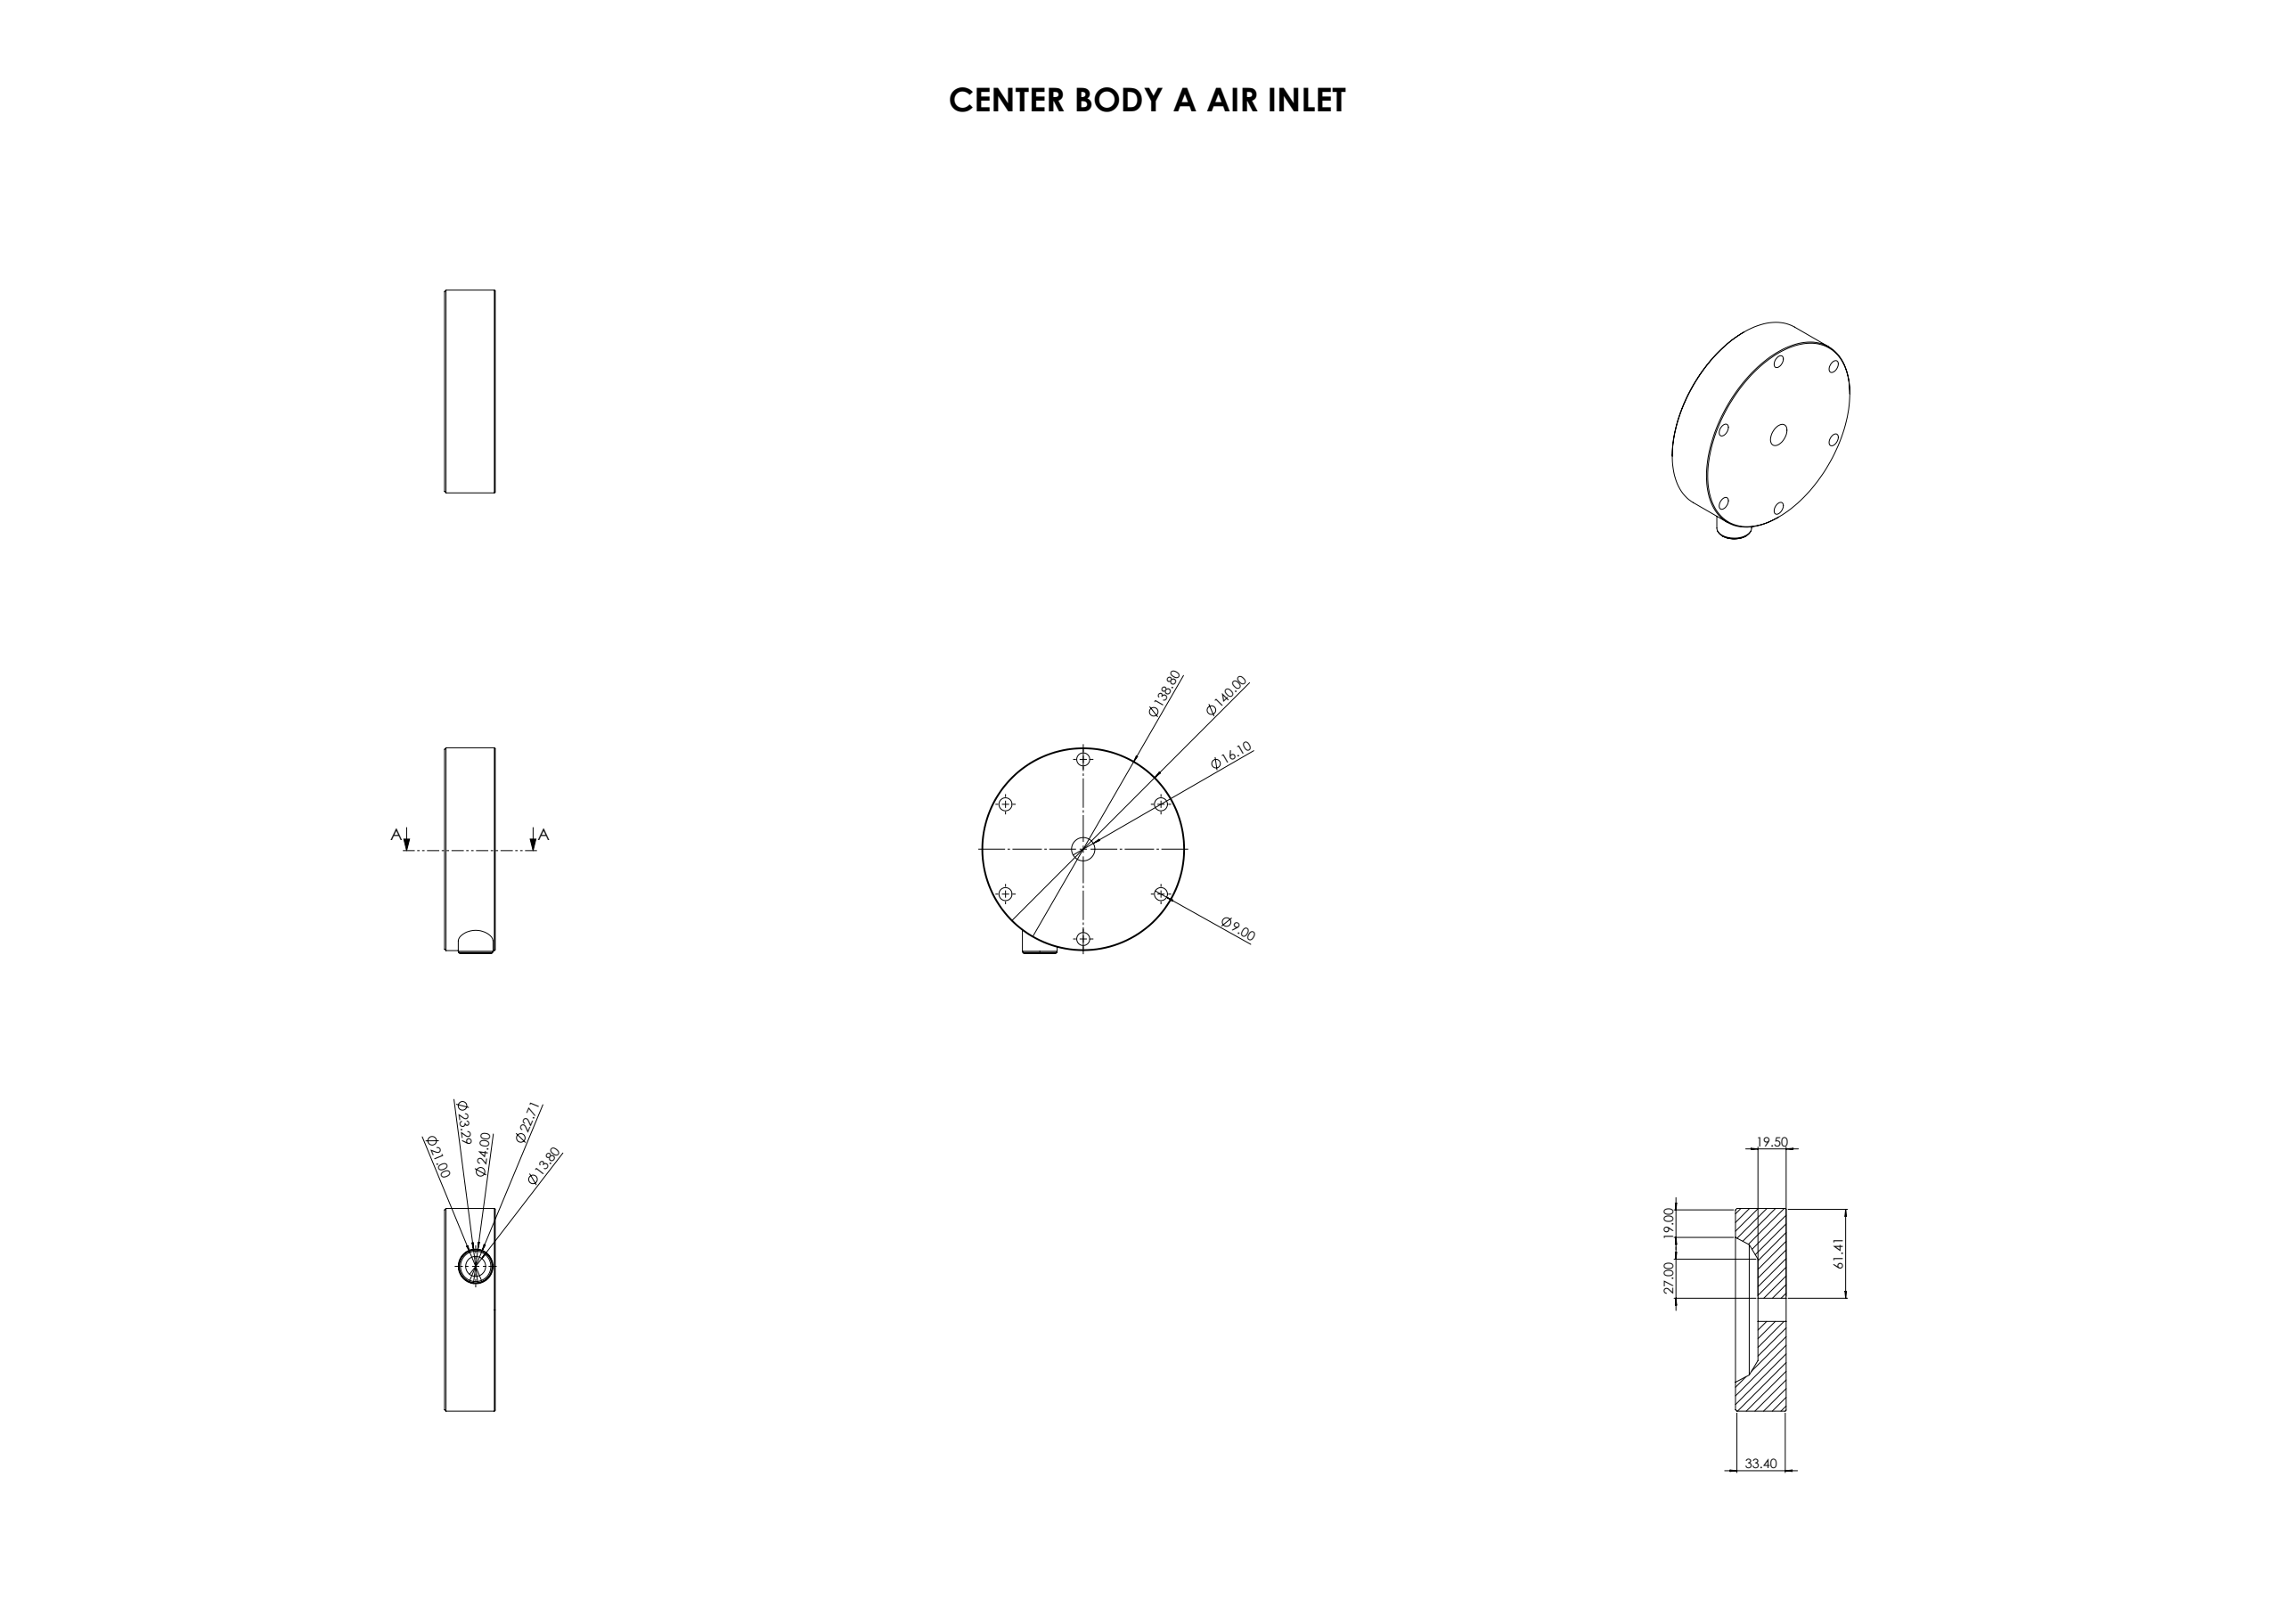
ISO-10303-21;
HEADER;
/* Generated by software containing ST-Developer
 * from STEP Tools, Inc. (www.steptools.com) 
 */

FILE_DESCRIPTION(
/* description */ (''),
/* implementation_level */ '2;1');

FILE_NAME(
/* name */ '02_Center_Body_A_Air_Inlet.step',
/* time_stamp */ '2026-10-26T06:13:19-07:00',
/* author */ (''),
/* organization */ (''),
/* preprocessor_version */ 'ST-DEVELOPER v20.2',
/* originating_system */ 'Autodesk Translation Framework v15.15.0.0',
/* authorisation */ '');

FILE_SCHEMA (('AUTOMOTIVE_DESIGN { 1 0 10303 214 3 1 1 }','TECHNICAL_DATA_PACKAGING'));
ENDSEC;

DATA;
#10=MECHANICAL_DESIGN_GEOMETRIC_PRESENTATION_REPRESENTATION('',(#298),#56639);
#258=SHAPE_REPRESENTATION_RELATIONSHIP('SRR','None',#56746,#278);
#278=ADVANCED_BREP_SHAPE_REPRESENTATION('',(#318),#56620);
#298=STYLED_ITEM('',(#56894),#318);
#318=MANIFOLD_SOLID_BREP('Body1',#16950);
#442=FACE_BOUND('',#2951,.T.);
#443=FACE_BOUND('',#2956,.T.);
#444=FACE_BOUND('',#2958,.T.);
#445=FACE_BOUND('',#2959,.T.);
#446=FACE_BOUND('',#2960,.T.);
#447=FACE_BOUND('',#2961,.T.);
#448=FACE_BOUND('',#2962,.T.);
#449=FACE_BOUND('',#2963,.T.);
#450=FACE_BOUND('',#2964,.T.);
#451=FACE_BOUND('',#2974,.T.);
#452=FACE_BOUND('',#2978,.T.);
#453=FACE_BOUND('',#2979,.T.);
#454=FACE_BOUND('',#2980,.T.);
#455=FACE_BOUND('',#2981,.T.);
#456=FACE_BOUND('',#2982,.T.);
#457=FACE_BOUND('',#2983,.T.);
#458=FACE_BOUND('',#2984,.T.);
#573=CONICAL_SURFACE('',#17486,10.9267766952966,1.17809724509617);
#574=CONICAL_SURFACE('',#17489,11.5,0.785398163397449);
#575=CONICAL_SURFACE('',#17493,11.8232233047034,0.392699081698727);
#576=CONICAL_SURFACE('',#17496,69.7,0.785398163397444);
#577=CONICAL_SURFACE('',#17528,40.,1.03037682652431);
#578=CONICAL_SURFACE('',#17530,47.5,0.484477929037023);
#579=CONICAL_SURFACE('',#17534,69.5,0.785398163397448);
#815=CIRCLE('',#17487,11.3535533905933);
#816=CIRCLE('',#17488,10.5);
#817=CIRCLE('',#17490,11.6464466094067);
#818=CIRCLE('',#17492,6.9);
#819=CIRCLE('',#17494,12.);
#820=CIRCLE('',#17497,69.4);
#821=CIRCLE('',#17498,70.);
#822=CIRCLE('',#17499,70.);
#823=CIRCLE('',#17501,70.);
#824=CIRCLE('',#17503,4.5);
#825=CIRCLE('',#17504,4.5);
#826=CIRCLE('',#17505,4.5);
#827=CIRCLE('',#17506,4.5);
#828=CIRCLE('',#17507,4.5);
#829=CIRCLE('',#17508,4.5);
#830=CIRCLE('',#17509,8.05);
#831=CIRCLE('',#17511,6.9);
#832=CIRCLE('',#17514,4.5);
#833=CIRCLE('',#17516,4.5);
#834=CIRCLE('',#17518,4.5);
#835=CIRCLE('',#17520,4.5);
#836=CIRCLE('',#17522,4.5);
#837=CIRCLE('',#17524,4.5);
#838=CIRCLE('',#17526,35.);
#839=CIRCLE('',#17527,8.05);
#840=CIRCLE('',#17529,45.);
#841=CIRCLE('',#17531,50.);
#842=CIRCLE('',#17533,69.);
#1281=CYLINDRICAL_SURFACE('',#17495,12.);
#1282=CYLINDRICAL_SURFACE('',#17500,70.);
#1283=CYLINDRICAL_SURFACE('',#17510,6.9);
#1284=CYLINDRICAL_SURFACE('',#17513,4.5);
#1285=CYLINDRICAL_SURFACE('',#17515,4.5);
#1286=CYLINDRICAL_SURFACE('',#17517,4.5);
#1287=CYLINDRICAL_SURFACE('',#17519,4.5);
#1288=CYLINDRICAL_SURFACE('',#17521,4.5);
#1289=CYLINDRICAL_SURFACE('',#17523,4.5);
#1290=CYLINDRICAL_SURFACE('',#17535,8.05);
#1947=FACE_OUTER_BOUND('',#2948,.T.);
#1948=FACE_OUTER_BOUND('',#2949,.T.);
#1949=FACE_OUTER_BOUND('',#2950,.T.);
#1950=FACE_OUTER_BOUND('',#2952,.T.);
#1951=FACE_OUTER_BOUND('',#2953,.T.);
#1952=FACE_OUTER_BOUND('',#2954,.T.);
#1953=FACE_OUTER_BOUND('',#2955,.T.);
#1954=FACE_OUTER_BOUND('',#2957,.T.);
#1955=FACE_OUTER_BOUND('',#2965,.T.);
#1956=FACE_OUTER_BOUND('',#2966,.T.);
#1957=FACE_OUTER_BOUND('',#2967,.T.);
#1958=FACE_OUTER_BOUND('',#2968,.T.);
#1959=FACE_OUTER_BOUND('',#2969,.T.);
#1960=FACE_OUTER_BOUND('',#2970,.T.);
#1961=FACE_OUTER_BOUND('',#2971,.T.);
#1962=FACE_OUTER_BOUND('',#2972,.T.);
#1963=FACE_OUTER_BOUND('',#2973,.T.);
#1964=FACE_OUTER_BOUND('',#2975,.T.);
#1965=FACE_OUTER_BOUND('',#2976,.T.);
#1966=FACE_OUTER_BOUND('',#2977,.T.);
#1967=FACE_OUTER_BOUND('',#2985,.T.);
#1968=FACE_OUTER_BOUND('',#2986,.T.);
#2948=EDGE_LOOP('',(#11496,#11497,#11498,#11499));
#2949=EDGE_LOOP('',(#11500,#11501,#11502,#11503));
#2950=EDGE_LOOP('',(#11504));
#2951=EDGE_LOOP('',(#11505));
#2952=EDGE_LOOP('',(#11506,#11507,#11508,#11509));
#2953=EDGE_LOOP('',(#11510,#11511,#11512,#11513,#11514));
#2954=EDGE_LOOP('',(#11515,#11516,#11517,#11518,#11519));
#2955=EDGE_LOOP('',(#11520,#11521,#11522,#11523,#11524));
#2956=EDGE_LOOP('',(#11525,#11526));
#2957=EDGE_LOOP('',(#11527));
#2958=EDGE_LOOP('',(#11528));
#2959=EDGE_LOOP('',(#11529));
#2960=EDGE_LOOP('',(#11530));
#2961=EDGE_LOOP('',(#11531));
#2962=EDGE_LOOP('',(#11532));
#2963=EDGE_LOOP('',(#11533));
#2964=EDGE_LOOP('',(#11534));
#2965=EDGE_LOOP('',(#11535,#11536,#11537,#11538));
#2966=EDGE_LOOP('',(#11539));
#2967=EDGE_LOOP('',(#11540,#11541,#11542,#11543));
#2968=EDGE_LOOP('',(#11544,#11545,#11546,#11547));
#2969=EDGE_LOOP('',(#11548,#11549,#11550,#11551));
#2970=EDGE_LOOP('',(#11552,#11553,#11554,#11555));
#2971=EDGE_LOOP('',(#11556,#11557,#11558,#11559));
#2972=EDGE_LOOP('',(#11560,#11561,#11562,#11563));
#2973=EDGE_LOOP('',(#11564));
#2974=EDGE_LOOP('',(#11565));
#2975=EDGE_LOOP('',(#11566,#11567,#11568,#11569));
#2976=EDGE_LOOP('',(#11570,#11571,#11572,#11573));
#2977=EDGE_LOOP('',(#11574));
#2978=EDGE_LOOP('',(#11575));
#2979=EDGE_LOOP('',(#11576));
#2980=EDGE_LOOP('',(#11577));
#2981=EDGE_LOOP('',(#11578));
#2982=EDGE_LOOP('',(#11579));
#2983=EDGE_LOOP('',(#11580));
#2984=EDGE_LOOP('',(#11581));
#2985=EDGE_LOOP('',(#11582,#11583,#11584,#11585));
#2986=EDGE_LOOP('',(#11586,#11587,#11588,#11589));
#4042=LINE('',#24660,#4996);
#4043=LINE('',#24664,#4997);
#4044=LINE('',#24671,#4998);
#4045=LINE('',#24675,#4999);
#4046=LINE('',#24721,#5000);
#4047=LINE('',#24727,#5001);
#4048=LINE('',#24746,#5002);
#4049=LINE('',#24751,#5003);
#4050=LINE('',#24755,#5004);
#4051=LINE('',#24759,#5005);
#4052=LINE('',#24763,#5006);
#4053=LINE('',#24767,#5007);
#4054=LINE('',#24771,#5008);
#4055=LINE('',#24780,#5009);
#4056=LINE('',#24784,#5010);
#4057=LINE('',#24790,#5011);
#4058=LINE('',#24792,#5012);
#4996=VECTOR('',#19526,10.9267766952966);
#4997=VECTOR('',#19531,11.5);
#4998=VECTOR('',#19540,11.8232233047034);
#4999=VECTOR('',#19545,12.);
#5000=VECTOR('',#19550,69.7);
#5001=VECTOR('',#19557,70.);
#5002=VECTOR('',#19578,6.9);
#5003=VECTOR('',#19585,4.5);
#5004=VECTOR('',#19590,4.5);
#5005=VECTOR('',#19595,4.5);
#5006=VECTOR('',#19600,4.5);
#5007=VECTOR('',#19605,4.5);
#5008=VECTOR('',#19610,4.5);
#5009=VECTOR('',#19621,40.);
#5010=VECTOR('',#19626,47.5);
#5011=VECTOR('',#19635,69.5);
#5012=VECTOR('',#19638,8.05);
#5877=B_SPLINE_CURVE_WITH_KNOTS('',3,(#24677,#24678,#24679,#24680,#24681,
#24682,#24683,#24684,#24685,#24686),.UNSPECIFIED.,.F.,.F.,(4,2,2,2,4),(0.,
0.449224301228608,0.898448602457216,1.38616749821439,1.87388639397155),
 .UNSPECIFIED.);
#5878=B_SPLINE_CURVE_WITH_KNOTS('',3,(#24687,#24688,#24689,#24690,#24691,
#24692,#24693,#24694,#24695,#24696,#24697,#24698,#24699,#24700,#24701,#24702,
#24703,#24704,#24705,#24706,#24707,#24708,#24709,#24710,#24711,#24712,#24713,
#24714,#24715,#24716),.UNSPECIFIED.,.F.,.F.,(4,2,2,2,2,2,2,2,2,2,2,2,2,
2,4),(1.87388639397155,2.39804133800567,2.92219628203978,3.37669912288026,
3.6039505433005,3.83120196372073,4.05845338414097,4.28570480456121,4.74020764540168,
5.2643625894358,5.78851753346991,6.27623642922708,6.76395532498425,7.21317962621286,
7.66240392744147),.UNSPECIFIED.);
#6943=VERTEX_POINT('',#24657);
#6944=VERTEX_POINT('',#24659);
#6945=VERTEX_POINT('',#24663);
#6946=VERTEX_POINT('',#24667);
#6947=VERTEX_POINT('',#24670);
#6948=VERTEX_POINT('',#24674);
#6949=VERTEX_POINT('',#24676);
#6950=VERTEX_POINT('',#24718);
#6951=VERTEX_POINT('',#24720);
#6952=VERTEX_POINT('',#24722);
#6953=VERTEX_POINT('',#24726);
#6954=VERTEX_POINT('',#24730);
#6955=VERTEX_POINT('',#24732);
#6956=VERTEX_POINT('',#24734);
#6957=VERTEX_POINT('',#24736);
#6958=VERTEX_POINT('',#24738);
#6959=VERTEX_POINT('',#24740);
#6960=VERTEX_POINT('',#24742);
#6961=VERTEX_POINT('',#24745);
#6962=VERTEX_POINT('',#24750);
#6963=VERTEX_POINT('',#24754);
#6964=VERTEX_POINT('',#24758);
#6965=VERTEX_POINT('',#24762);
#6966=VERTEX_POINT('',#24766);
#6967=VERTEX_POINT('',#24770);
#6968=VERTEX_POINT('',#24774);
#6969=VERTEX_POINT('',#24776);
#6970=VERTEX_POINT('',#24779);
#6971=VERTEX_POINT('',#24783);
#6972=VERTEX_POINT('',#24787);
#8655=EDGE_CURVE('',#6943,#6943,#815,.T.);
#8656=EDGE_CURVE('',#6943,#6944,#4042,.T.);
#8657=EDGE_CURVE('',#6944,#6944,#816,.T.);
#8658=EDGE_CURVE('',#6943,#6945,#4043,.T.);
#8659=EDGE_CURVE('',#6945,#6945,#817,.T.);
#8660=EDGE_CURVE('',#6946,#6946,#818,.T.);
#8661=EDGE_CURVE('',#6945,#6947,#4044,.T.);
#8662=EDGE_CURVE('',#6947,#6947,#819,.T.);
#8663=EDGE_CURVE('',#6947,#6948,#4045,.T.);
#8664=EDGE_CURVE('',#6949,#6948,#5877,.T.);
#8665=EDGE_CURVE('',#6948,#6949,#5878,.T.);
#8666=EDGE_CURVE('',#6950,#6950,#820,.T.);
#8667=EDGE_CURVE('',#6950,#6951,#4046,.T.);
#8668=EDGE_CURVE('',#6951,#6952,#821,.T.);
#8669=EDGE_CURVE('',#6952,#6951,#822,.T.);
#8670=EDGE_CURVE('',#6952,#6953,#4047,.T.);
#8671=EDGE_CURVE('',#6953,#6953,#823,.T.);
#8672=EDGE_CURVE('',#6954,#6954,#824,.T.);
#8673=EDGE_CURVE('',#6955,#6955,#825,.T.);
#8674=EDGE_CURVE('',#6956,#6956,#826,.T.);
#8675=EDGE_CURVE('',#6957,#6957,#827,.T.);
#8676=EDGE_CURVE('',#6958,#6958,#828,.T.);
#8677=EDGE_CURVE('',#6959,#6959,#829,.T.);
#8678=EDGE_CURVE('',#6960,#6960,#830,.T.);
#8679=EDGE_CURVE('',#6946,#6961,#4048,.T.);
#8680=EDGE_CURVE('',#6961,#6961,#831,.T.);
#8681=EDGE_CURVE('',#6954,#6962,#4049,.T.);
#8682=EDGE_CURVE('',#6962,#6962,#832,.T.);
#8683=EDGE_CURVE('',#6955,#6963,#4050,.T.);
#8684=EDGE_CURVE('',#6963,#6963,#833,.T.);
#8685=EDGE_CURVE('',#6956,#6964,#4051,.T.);
#8686=EDGE_CURVE('',#6964,#6964,#834,.T.);
#8687=EDGE_CURVE('',#6957,#6965,#4052,.T.);
#8688=EDGE_CURVE('',#6965,#6965,#835,.T.);
#8689=EDGE_CURVE('',#6958,#6966,#4053,.T.);
#8690=EDGE_CURVE('',#6966,#6966,#836,.T.);
#8691=EDGE_CURVE('',#6959,#6967,#4054,.T.);
#8692=EDGE_CURVE('',#6967,#6967,#837,.T.);
#8693=EDGE_CURVE('',#6968,#6968,#838,.T.);
#8694=EDGE_CURVE('',#6969,#6969,#839,.T.);
#8695=EDGE_CURVE('',#6968,#6970,#4055,.T.);
#8696=EDGE_CURVE('',#6970,#6970,#840,.T.);
#8697=EDGE_CURVE('',#6970,#6971,#4056,.T.);
#8698=EDGE_CURVE('',#6971,#6971,#841,.T.);
#8699=EDGE_CURVE('',#6972,#6972,#842,.T.);
#8700=EDGE_CURVE('',#6953,#6972,#4057,.T.);
#8701=EDGE_CURVE('',#6960,#6969,#4058,.T.);
#11496=ORIENTED_EDGE('',*,*,#8655,.T.);
#11497=ORIENTED_EDGE('',*,*,#8656,.T.);
#11498=ORIENTED_EDGE('',*,*,#8657,.T.);
#11499=ORIENTED_EDGE('',*,*,#8656,.F.);
#11500=ORIENTED_EDGE('',*,*,#8655,.F.);
#11501=ORIENTED_EDGE('',*,*,#8658,.T.);
#11502=ORIENTED_EDGE('',*,*,#8659,.F.);
#11503=ORIENTED_EDGE('',*,*,#8658,.F.);
#11504=ORIENTED_EDGE('',*,*,#8657,.F.);
#11505=ORIENTED_EDGE('',*,*,#8660,.T.);
#11506=ORIENTED_EDGE('',*,*,#8659,.T.);
#11507=ORIENTED_EDGE('',*,*,#8661,.T.);
#11508=ORIENTED_EDGE('',*,*,#8662,.T.);
#11509=ORIENTED_EDGE('',*,*,#8661,.F.);
#11510=ORIENTED_EDGE('',*,*,#8662,.F.);
#11511=ORIENTED_EDGE('',*,*,#8663,.T.);
#11512=ORIENTED_EDGE('',*,*,#8664,.F.);
#11513=ORIENTED_EDGE('',*,*,#8665,.F.);
#11514=ORIENTED_EDGE('',*,*,#8663,.F.);
#11515=ORIENTED_EDGE('',*,*,#8666,.T.);
#11516=ORIENTED_EDGE('',*,*,#8667,.T.);
#11517=ORIENTED_EDGE('',*,*,#8668,.T.);
#11518=ORIENTED_EDGE('',*,*,#8669,.T.);
#11519=ORIENTED_EDGE('',*,*,#8667,.F.);
#11520=ORIENTED_EDGE('',*,*,#8668,.F.);
#11521=ORIENTED_EDGE('',*,*,#8669,.F.);
#11522=ORIENTED_EDGE('',*,*,#8670,.T.);
#11523=ORIENTED_EDGE('',*,*,#8671,.T.);
#11524=ORIENTED_EDGE('',*,*,#8670,.F.);
#11525=ORIENTED_EDGE('',*,*,#8664,.T.);
#11526=ORIENTED_EDGE('',*,*,#8665,.T.);
#11527=ORIENTED_EDGE('',*,*,#8666,.F.);
#11528=ORIENTED_EDGE('',*,*,#8672,.T.);
#11529=ORIENTED_EDGE('',*,*,#8673,.T.);
#11530=ORIENTED_EDGE('',*,*,#8674,.T.);
#11531=ORIENTED_EDGE('',*,*,#8675,.T.);
#11532=ORIENTED_EDGE('',*,*,#8676,.T.);
#11533=ORIENTED_EDGE('',*,*,#8677,.T.);
#11534=ORIENTED_EDGE('',*,*,#8678,.F.);
#11535=ORIENTED_EDGE('',*,*,#8660,.F.);
#11536=ORIENTED_EDGE('',*,*,#8679,.T.);
#11537=ORIENTED_EDGE('',*,*,#8680,.T.);
#11538=ORIENTED_EDGE('',*,*,#8679,.F.);
#11539=ORIENTED_EDGE('',*,*,#8680,.F.);
#11540=ORIENTED_EDGE('',*,*,#8672,.F.);
#11541=ORIENTED_EDGE('',*,*,#8681,.T.);
#11542=ORIENTED_EDGE('',*,*,#8682,.F.);
#11543=ORIENTED_EDGE('',*,*,#8681,.F.);
#11544=ORIENTED_EDGE('',*,*,#8673,.F.);
#11545=ORIENTED_EDGE('',*,*,#8683,.T.);
#11546=ORIENTED_EDGE('',*,*,#8684,.F.);
#11547=ORIENTED_EDGE('',*,*,#8683,.F.);
#11548=ORIENTED_EDGE('',*,*,#8674,.F.);
#11549=ORIENTED_EDGE('',*,*,#8685,.T.);
#11550=ORIENTED_EDGE('',*,*,#8686,.F.);
#11551=ORIENTED_EDGE('',*,*,#8685,.F.);
#11552=ORIENTED_EDGE('',*,*,#8675,.F.);
#11553=ORIENTED_EDGE('',*,*,#8687,.T.);
#11554=ORIENTED_EDGE('',*,*,#8688,.F.);
#11555=ORIENTED_EDGE('',*,*,#8687,.F.);
#11556=ORIENTED_EDGE('',*,*,#8676,.F.);
#11557=ORIENTED_EDGE('',*,*,#8689,.T.);
#11558=ORIENTED_EDGE('',*,*,#8690,.F.);
#11559=ORIENTED_EDGE('',*,*,#8689,.F.);
#11560=ORIENTED_EDGE('',*,*,#8677,.F.);
#11561=ORIENTED_EDGE('',*,*,#8691,.T.);
#11562=ORIENTED_EDGE('',*,*,#8692,.F.);
#11563=ORIENTED_EDGE('',*,*,#8691,.F.);
#11564=ORIENTED_EDGE('',*,*,#8693,.F.);
#11565=ORIENTED_EDGE('',*,*,#8694,.T.);
#11566=ORIENTED_EDGE('',*,*,#8693,.T.);
#11567=ORIENTED_EDGE('',*,*,#8695,.T.);
#11568=ORIENTED_EDGE('',*,*,#8696,.F.);
#11569=ORIENTED_EDGE('',*,*,#8695,.F.);
#11570=ORIENTED_EDGE('',*,*,#8696,.T.);
#11571=ORIENTED_EDGE('',*,*,#8697,.T.);
#11572=ORIENTED_EDGE('',*,*,#8698,.F.);
#11573=ORIENTED_EDGE('',*,*,#8697,.F.);
#11574=ORIENTED_EDGE('',*,*,#8699,.F.);
#11575=ORIENTED_EDGE('',*,*,#8698,.T.);
#11576=ORIENTED_EDGE('',*,*,#8692,.T.);
#11577=ORIENTED_EDGE('',*,*,#8690,.T.);
#11578=ORIENTED_EDGE('',*,*,#8688,.T.);
#11579=ORIENTED_EDGE('',*,*,#8686,.T.);
#11580=ORIENTED_EDGE('',*,*,#8684,.T.);
#11581=ORIENTED_EDGE('',*,*,#8682,.T.);
#11582=ORIENTED_EDGE('',*,*,#8671,.F.);
#11583=ORIENTED_EDGE('',*,*,#8700,.T.);
#11584=ORIENTED_EDGE('',*,*,#8699,.T.);
#11585=ORIENTED_EDGE('',*,*,#8700,.F.);
#11586=ORIENTED_EDGE('',*,*,#8678,.T.);
#11587=ORIENTED_EDGE('',*,*,#8701,.T.);
#11588=ORIENTED_EDGE('',*,*,#8694,.F.);
#11589=ORIENTED_EDGE('',*,*,#8701,.F.);
#15763=PLANE('',#17491);
#15764=PLANE('',#17502);
#15765=PLANE('',#17512);
#15766=PLANE('',#17525);
#15767=PLANE('',#17532);
#16118=ADVANCED_FACE('',(#1947),#573,.T.);
#16119=ADVANCED_FACE('',(#1948),#574,.T.);
#16120=ADVANCED_FACE('',(#1949,#442),#15763,.F.);
#16121=ADVANCED_FACE('',(#1950),#575,.T.);
#16122=ADVANCED_FACE('',(#1951),#1281,.T.);
#16123=ADVANCED_FACE('',(#1952),#576,.T.);
#16124=ADVANCED_FACE('',(#1953,#443),#1282,.T.);
#16125=ADVANCED_FACE('',(#1954,#444,#445,#446,#447,#448,#449,#450),#15764,
 .T.);
#16126=ADVANCED_FACE('',(#1955),#1283,.F.);
#16127=ADVANCED_FACE('',(#1956),#15765,.F.);
#16128=ADVANCED_FACE('',(#1957),#1284,.F.);
#16129=ADVANCED_FACE('',(#1958),#1285,.F.);
#16130=ADVANCED_FACE('',(#1959),#1286,.F.);
#16131=ADVANCED_FACE('',(#1960),#1287,.F.);
#16132=ADVANCED_FACE('',(#1961),#1288,.F.);
#16133=ADVANCED_FACE('',(#1962),#1289,.F.);
#16134=ADVANCED_FACE('',(#1963,#451),#15766,.T.);
#16135=ADVANCED_FACE('',(#1964),#577,.F.);
#16136=ADVANCED_FACE('',(#1965),#578,.F.);
#16137=ADVANCED_FACE('',(#1966,#452,#453,#454,#455,#456,#457,#458),#15767,
 .T.);
#16138=ADVANCED_FACE('',(#1967),#579,.T.);
#16139=ADVANCED_FACE('',(#1968),#1290,.F.);
#16950=CLOSED_SHELL('',(#16118,#16119,#16120,#16121,#16122,#16123,#16124,
#16125,#16126,#16127,#16128,#16129,#16130,#16131,#16132,#16133,#16134,#16135,
#16136,#16137,#16138,#16139));
#17485=AXIS2_PLACEMENT_3D('',#24655,#19520,#19521);
#17486=AXIS2_PLACEMENT_3D('',#24656,#19522,#19523);
#17487=AXIS2_PLACEMENT_3D('',#24658,#19524,#19525);
#17488=AXIS2_PLACEMENT_3D('',#24661,#19527,#19528);
#17489=AXIS2_PLACEMENT_3D('',#24662,#19529,#19530);
#17490=AXIS2_PLACEMENT_3D('',#24665,#19532,#19533);
#17491=AXIS2_PLACEMENT_3D('',#24666,#19534,#19535);
#17492=AXIS2_PLACEMENT_3D('',#24668,#19536,#19537);
#17493=AXIS2_PLACEMENT_3D('',#24669,#19538,#19539);
#17494=AXIS2_PLACEMENT_3D('',#24672,#19541,#19542);
#17495=AXIS2_PLACEMENT_3D('',#24673,#19543,#19544);
#17496=AXIS2_PLACEMENT_3D('',#24717,#19546,#19547);
#17497=AXIS2_PLACEMENT_3D('',#24719,#19548,#19549);
#17498=AXIS2_PLACEMENT_3D('',#24723,#19551,#19552);
#17499=AXIS2_PLACEMENT_3D('',#24724,#19553,#19554);
#17500=AXIS2_PLACEMENT_3D('',#24725,#19555,#19556);
#17501=AXIS2_PLACEMENT_3D('',#24728,#19558,#19559);
#17502=AXIS2_PLACEMENT_3D('',#24729,#19560,#19561);
#17503=AXIS2_PLACEMENT_3D('',#24731,#19562,#19563);
#17504=AXIS2_PLACEMENT_3D('',#24733,#19564,#19565);
#17505=AXIS2_PLACEMENT_3D('',#24735,#19566,#19567);
#17506=AXIS2_PLACEMENT_3D('',#24737,#19568,#19569);
#17507=AXIS2_PLACEMENT_3D('',#24739,#19570,#19571);
#17508=AXIS2_PLACEMENT_3D('',#24741,#19572,#19573);
#17509=AXIS2_PLACEMENT_3D('',#24743,#19574,#19575);
#17510=AXIS2_PLACEMENT_3D('',#24744,#19576,#19577);
#17511=AXIS2_PLACEMENT_3D('',#24747,#19579,#19580);
#17512=AXIS2_PLACEMENT_3D('',#24748,#19581,#19582);
#17513=AXIS2_PLACEMENT_3D('',#24749,#19583,#19584);
#17514=AXIS2_PLACEMENT_3D('',#24752,#19586,#19587);
#17515=AXIS2_PLACEMENT_3D('',#24753,#19588,#19589);
#17516=AXIS2_PLACEMENT_3D('',#24756,#19591,#19592);
#17517=AXIS2_PLACEMENT_3D('',#24757,#19593,#19594);
#17518=AXIS2_PLACEMENT_3D('',#24760,#19596,#19597);
#17519=AXIS2_PLACEMENT_3D('',#24761,#19598,#19599);
#17520=AXIS2_PLACEMENT_3D('',#24764,#19601,#19602);
#17521=AXIS2_PLACEMENT_3D('',#24765,#19603,#19604);
#17522=AXIS2_PLACEMENT_3D('',#24768,#19606,#19607);
#17523=AXIS2_PLACEMENT_3D('',#24769,#19608,#19609);
#17524=AXIS2_PLACEMENT_3D('',#24772,#19611,#19612);
#17525=AXIS2_PLACEMENT_3D('',#24773,#19613,#19614);
#17526=AXIS2_PLACEMENT_3D('',#24775,#19615,#19616);
#17527=AXIS2_PLACEMENT_3D('',#24777,#19617,#19618);
#17528=AXIS2_PLACEMENT_3D('',#24778,#19619,#19620);
#17529=AXIS2_PLACEMENT_3D('',#24781,#19622,#19623);
#17530=AXIS2_PLACEMENT_3D('',#24782,#19624,#19625);
#17531=AXIS2_PLACEMENT_3D('',#24785,#19627,#19628);
#17532=AXIS2_PLACEMENT_3D('',#24786,#19629,#19630);
#17533=AXIS2_PLACEMENT_3D('',#24788,#19631,#19632);
#17534=AXIS2_PLACEMENT_3D('',#24789,#19633,#19634);
#17535=AXIS2_PLACEMENT_3D('',#24791,#19636,#19637);
#19520=DIRECTION('axis',(0.,0.,1.));
#19521=DIRECTION('refdir',(1.,0.,0.));
#19522=DIRECTION('center_axis',(0.,1.,0.));
#19523=DIRECTION('ref_axis',(1.,0.,0.));
#19524=DIRECTION('center_axis',(0.,-1.,0.));
#19525=DIRECTION('ref_axis',(1.,0.,0.));
#19526=DIRECTION('',(0.923879532511287,-0.38268343236509,-1.1314261122877E-16));
#19527=DIRECTION('center_axis',(0.,1.,0.));
#19528=DIRECTION('ref_axis',(1.,0.,0.));
#19529=DIRECTION('center_axis',(0.,1.,0.));
#19530=DIRECTION('ref_axis',(1.,0.,0.));
#19531=DIRECTION('',(-0.707106781186548,0.707106781186547,-8.65956056235494E-17));
#19532=DIRECTION('center_axis',(0.,1.,0.));
#19533=DIRECTION('ref_axis',(1.,0.,0.));
#19534=DIRECTION('center_axis',(0.,1.,0.));
#19535=DIRECTION('ref_axis',(1.,0.,0.));
#19536=DIRECTION('center_axis',(0.,1.,0.));
#19537=DIRECTION('ref_axis',(1.,0.,0.));
#19538=DIRECTION('center_axis',(0.,1.,0.));
#19539=DIRECTION('ref_axis',(1.,0.,0.));
#19540=DIRECTION('',(-0.382683432365092,0.923879532511286,-4.68652040532633E-17));
#19541=DIRECTION('center_axis',(0.,-1.,0.));
#19542=DIRECTION('ref_axis',(1.,0.,0.));
#19543=DIRECTION('center_axis',(0.,-1.,0.));
#19544=DIRECTION('ref_axis',(1.,0.,0.));
#19545=DIRECTION('',(0.,1.,0.));
#19546=DIRECTION('center_axis',(-1.,0.,0.));
#19547=DIRECTION('ref_axis',(0.,-1.,0.));
#19548=DIRECTION('center_axis',(-1.,0.,0.));
#19549=DIRECTION('ref_axis',(0.,-1.,0.));
#19550=DIRECTION('',(-0.70710678118655,0.707106781186545,8.6595605623549E-17));
#19551=DIRECTION('center_axis',(1.,0.,0.));
#19552=DIRECTION('ref_axis',(0.,-1.,0.));
#19553=DIRECTION('center_axis',(1.,0.,0.));
#19554=DIRECTION('ref_axis',(0.,-1.,0.));
#19555=DIRECTION('center_axis',(1.,0.,0.));
#19556=DIRECTION('ref_axis',(0.,1.,0.));
#19557=DIRECTION('',(-1.,0.,0.));
#19558=DIRECTION('center_axis',(1.,0.,0.));
#19559=DIRECTION('ref_axis',(0.,0.,-1.));
#19560=DIRECTION('center_axis',(1.,0.,0.));
#19561=DIRECTION('ref_axis',(0.,0.,-1.));
#19562=DIRECTION('center_axis',(-1.,0.,0.));
#19563=DIRECTION('ref_axis',(0.,0.,-1.));
#19564=DIRECTION('center_axis',(-1.,0.,0.));
#19565=DIRECTION('ref_axis',(0.,0.,-1.));
#19566=DIRECTION('center_axis',(-1.,0.,0.));
#19567=DIRECTION('ref_axis',(0.,0.,-1.));
#19568=DIRECTION('center_axis',(-1.,0.,0.));
#19569=DIRECTION('ref_axis',(0.,0.,-1.));
#19570=DIRECTION('center_axis',(-1.,0.,0.));
#19571=DIRECTION('ref_axis',(0.,0.,-1.));
#19572=DIRECTION('center_axis',(-1.,0.,0.));
#19573=DIRECTION('ref_axis',(0.,0.,-1.));
#19574=DIRECTION('center_axis',(1.,0.,0.));
#19575=DIRECTION('ref_axis',(0.,0.,-1.));
#19576=DIRECTION('center_axis',(0.,1.,0.));
#19577=DIRECTION('ref_axis',(1.,0.,0.));
#19578=DIRECTION('',(0.,1.,0.));
#19579=DIRECTION('center_axis',(0.,1.,0.));
#19580=DIRECTION('ref_axis',(1.,0.,0.));
#19581=DIRECTION('center_axis',(0.,1.,0.));
#19582=DIRECTION('ref_axis',(1.,0.,0.));
#19583=DIRECTION('center_axis',(-1.,0.,0.));
#19584=DIRECTION('ref_axis',(0.,0.,-1.));
#19585=DIRECTION('',(-1.,0.,0.));
#19586=DIRECTION('center_axis',(1.,0.,0.));
#19587=DIRECTION('ref_axis',(0.,0.,-1.));
#19588=DIRECTION('center_axis',(-1.,0.,0.));
#19589=DIRECTION('ref_axis',(0.,0.,-1.));
#19590=DIRECTION('',(-1.,0.,0.));
#19591=DIRECTION('center_axis',(1.,0.,0.));
#19592=DIRECTION('ref_axis',(0.,0.,-1.));
#19593=DIRECTION('center_axis',(-1.,0.,0.));
#19594=DIRECTION('ref_axis',(0.,0.,-1.));
#19595=DIRECTION('',(-1.,0.,0.));
#19596=DIRECTION('center_axis',(1.,0.,0.));
#19597=DIRECTION('ref_axis',(0.,0.,-1.));
#19598=DIRECTION('center_axis',(-1.,0.,0.));
#19599=DIRECTION('ref_axis',(0.,0.,-1.));
#19600=DIRECTION('',(-1.,0.,0.));
#19601=DIRECTION('center_axis',(1.,0.,0.));
#19602=DIRECTION('ref_axis',(0.,0.,-1.));
#19603=DIRECTION('center_axis',(-1.,0.,0.));
#19604=DIRECTION('ref_axis',(0.,0.,-1.));
#19605=DIRECTION('',(-1.,0.,0.));
#19606=DIRECTION('center_axis',(1.,0.,0.));
#19607=DIRECTION('ref_axis',(0.,0.,-1.));
#19608=DIRECTION('center_axis',(-1.,0.,0.));
#19609=DIRECTION('ref_axis',(0.,0.,-1.));
#19610=DIRECTION('',(-1.,0.,0.));
#19611=DIRECTION('center_axis',(1.,0.,0.));
#19612=DIRECTION('ref_axis',(0.,0.,-1.));
#19613=DIRECTION('center_axis',(-1.,0.,0.));
#19614=DIRECTION('ref_axis',(0.,0.,1.));
#19615=DIRECTION('center_axis',(1.,0.,0.));
#19616=DIRECTION('ref_axis',(0.,0.,-1.));
#19617=DIRECTION('center_axis',(1.,0.,0.));
#19618=DIRECTION('ref_axis',(0.,0.,-1.));
#19619=DIRECTION('center_axis',(-1.,0.,0.));
#19620=DIRECTION('ref_axis',(0.,1.,0.));
#19621=DIRECTION('',(-0.514495755427527,-0.857492925712544,-1.05012596676537E-16));
#19622=DIRECTION('center_axis',(1.,0.,0.));
#19623=DIRECTION('ref_axis',(0.,0.,-1.));
#19624=DIRECTION('center_axis',(-1.,0.,0.));
#19625=DIRECTION('ref_axis',(0.,1.,0.));
#19626=DIRECTION('',(-0.884918222381982,-0.465746432832622,-5.70374878182769E-17));
#19627=DIRECTION('center_axis',(1.,0.,0.));
#19628=DIRECTION('ref_axis',(0.,0.,-1.));
#19629=DIRECTION('center_axis',(-1.,0.,0.));
#19630=DIRECTION('ref_axis',(0.,0.,1.));
#19631=DIRECTION('center_axis',(1.,0.,0.));
#19632=DIRECTION('ref_axis',(0.,0.,-1.));
#19633=DIRECTION('center_axis',(1.,0.,0.));
#19634=DIRECTION('ref_axis',(0.,1.,0.));
#19635=DIRECTION('',(-0.707106781186547,0.707106781186547,8.65956056235493E-17));
#19636=DIRECTION('center_axis',(1.,0.,0.));
#19637=DIRECTION('ref_axis',(0.,1.,0.));
#19638=DIRECTION('',(-1.,0.,0.));
#24655=CARTESIAN_POINT('',(0.,0.,0.));
#24656=CARTESIAN_POINT('Origin',(-14.,-71.8232233047034,30.));
#24657=CARTESIAN_POINT('',(-25.3535533905933,-71.6464466094067,30.));
#24658=CARTESIAN_POINT('Origin',(-14.,-71.6464466094067,30.));
#24659=CARTESIAN_POINT('',(-24.5,-72.,30.));
#24660=CARTESIAN_POINT('',(-24.9267766952966,-71.8232233047034,30.));
#24661=CARTESIAN_POINT('Origin',(-14.,-72.,30.));
#24662=CARTESIAN_POINT('Origin',(-14.,-71.5,30.));
#24663=CARTESIAN_POINT('',(-25.6464466094067,-71.3535533905933,30.));
#24664=CARTESIAN_POINT('',(-25.5,-71.5,30.));
#24665=CARTESIAN_POINT('Origin',(-14.,-71.3535533905933,30.));
#24666=CARTESIAN_POINT('Origin',(-14.,-72.,30.));
#24667=CARTESIAN_POINT('',(-20.9,-72.,30.));
#24668=CARTESIAN_POINT('Origin',(-14.,-72.,30.));
#24669=CARTESIAN_POINT('Origin',(-14.,-70.9267766952966,30.));
#24670=CARTESIAN_POINT('',(-26.,-70.5,30.));
#24671=CARTESIAN_POINT('',(-25.8232233047034,-70.9267766952966,30.));
#24672=CARTESIAN_POINT('Origin',(-14.,-70.5,30.));
#24673=CARTESIAN_POINT('Origin',(-14.,-50.,30.));
#24674=CARTESIAN_POINT('',(-26.,-63.2455532033676,30.));
#24675=CARTESIAN_POINT('',(-26.,-50.,30.));
#24676=CARTESIAN_POINT('',(-14.,-67.6461381011511,18.));
#24677=CARTESIAN_POINT('Ctrl Pts',(-14.,-67.6461381011511,18.));
#24678=CARTESIAN_POINT('Ctrl Pts',(-15.4974143374287,-67.6461381011511,
18.));
#24679=CARTESIAN_POINT('Ctrl Pts',(-17.0915205041766,-67.569001302991,18.2980124136255));
#24680=CARTESIAN_POINT('Ctrl Pts',(-20.0138657590624,-67.2330346371868,
19.4963139645897));
#24681=CARTESIAN_POINT('Ctrl Pts',(-21.3418872514445,-66.9712006520621,
20.3962895865205));
#24682=CARTESIAN_POINT('Ctrl Pts',(-23.5213138818415,-66.2867646794087,
22.5260020891911));
#24683=CARTESIAN_POINT('Ctrl Pts',(-24.4747045274443,-65.8046030416515,
23.9238828818556));
#24684=CARTESIAN_POINT('Ctrl Pts',(-25.713131811207,-64.6337042024678,26.9273511571404));
#24685=CARTESIAN_POINT('Ctrl Pts',(-26.,-63.9422944830207,28.5311404109572));
#24686=CARTESIAN_POINT('Ctrl Pts',(-26.,-63.2455532033676,30.));
#24687=CARTESIAN_POINT('Ctrl Pts',(-26.,-63.2455532033676,30.));
#24688=CARTESIAN_POINT('Ctrl Pts',(-26.,-62.496760426176,31.5785937809389));
#24689=CARTESIAN_POINT('Ctrl Pts',(-25.6727630693155,-61.6315633847307,
33.2354648264254));
#24690=CARTESIAN_POINT('Ctrl Pts',(-24.366604146322,-59.898806525139,36.2653926472075));
#24691=CARTESIAN_POINT('Ctrl Pts',(-23.3890813807094,-59.033283877067,37.6402168655692));
#24692=CARTESIAN_POINT('Ctrl Pts',(-21.2292573598961,-57.6805770802603,
39.6766954896892));
#24693=CARTESIAN_POINT('Ctrl Pts',(-19.952736536109,-57.0753995031866,40.5328837235444));
#24694=CARTESIAN_POINT('Ctrl Pts',(-17.8109551249349,-56.4425965862802,
41.4048580623199));
#24695=CARTESIAN_POINT('Ctrl Pts',(-17.0595209591031,-56.2763096504852,
41.6294531705792));
#24696=CARTESIAN_POINT('Ctrl Pts',(-15.5328204392415,-56.0549204173022,
41.9270830875605));
#24697=CARTESIAN_POINT('Ctrl Pts',(-14.7575047347341,-56.,42.));
#24698=CARTESIAN_POINT('Ctrl Pts',(-13.2424952652659,-56.,42.));
#24699=CARTESIAN_POINT('Ctrl Pts',(-12.4671795607585,-56.0549204173022,
41.9270830875605));
#24700=CARTESIAN_POINT('Ctrl Pts',(-10.9404790408969,-56.2763096504852,
41.6294531705792));
#24701=CARTESIAN_POINT('Ctrl Pts',(-10.1890448750651,-56.4425965862802,
41.4048580623199));
#24702=CARTESIAN_POINT('Ctrl Pts',(-8.04726346389096,-57.0753995031866,
40.5328837235444));
#24703=CARTESIAN_POINT('Ctrl Pts',(-6.77074264010388,-57.6805770802603,
39.6766954896892));
#24704=CARTESIAN_POINT('Ctrl Pts',(-4.61091861929063,-59.033283877067,37.6402168655692));
#24705=CARTESIAN_POINT('Ctrl Pts',(-3.63339585367803,-59.898806525139,36.2653926472075));
#24706=CARTESIAN_POINT('Ctrl Pts',(-2.32723693068453,-61.6315633847307,
33.2354648264254));
#24707=CARTESIAN_POINT('Ctrl Pts',(-2.,-62.496760426176,31.578593780939));
#24708=CARTESIAN_POINT('Ctrl Pts',(-2.,-63.9422944830207,28.5311404109573));
#24709=CARTESIAN_POINT('Ctrl Pts',(-2.28686818879297,-64.6337042024678,
26.9273511571404));
#24710=CARTESIAN_POINT('Ctrl Pts',(-3.52529547255565,-65.8046030416515,
23.9238828818556));
#24711=CARTESIAN_POINT('Ctrl Pts',(-4.47868611815846,-66.2867646794087,
22.5260020891911));
#24712=CARTESIAN_POINT('Ctrl Pts',(-6.65811274855545,-66.9712006520621,
20.3962895865205));
#24713=CARTESIAN_POINT('Ctrl Pts',(-7.98613424093757,-67.2330346371868,
19.4963139645897));
#24714=CARTESIAN_POINT('Ctrl Pts',(-10.9084794958234,-67.569001302991,18.2980124136255));
#24715=CARTESIAN_POINT('Ctrl Pts',(-12.5025856625713,-67.6461381011511,
18.));
#24716=CARTESIAN_POINT('Ctrl Pts',(-14.,-67.6461381011511,18.));
#24717=CARTESIAN_POINT('Origin',(-0.8,0.,0.));
#24718=CARTESIAN_POINT('',(-0.5,69.4,-8.49904878608263E-15));
#24719=CARTESIAN_POINT('Origin',(-0.5,0.,0.));
#24720=CARTESIAN_POINT('',(-1.1,70.,8.57252759403147E-15));
#24721=CARTESIAN_POINT('',(-0.8,69.7,8.53578819005705E-15));
#24722=CARTESIAN_POINT('',(-1.1,-70.,-8.57252759403147E-15));
#24723=CARTESIAN_POINT('Origin',(-1.1,0.,0.));
#24724=CARTESIAN_POINT('Origin',(-1.1,0.,0.));
#24725=CARTESIAN_POINT('Origin',(-17.5,0.,0.));
#24726=CARTESIAN_POINT('',(-34.5,-70.,-8.57252759403147E-15));
#24727=CARTESIAN_POINT('',(-17.5,-70.,-8.57252759403147E-15));
#24728=CARTESIAN_POINT('Origin',(-34.5,0.,0.));
#24729=CARTESIAN_POINT('Origin',(-0.5,8.05,0.));
#24730=CARTESIAN_POINT('',(-0.5,-31.,-49.1935750346352));
#24731=CARTESIAN_POINT('Origin',(-0.5,-31.,-53.6935750346352));
#24732=CARTESIAN_POINT('',(-0.5,62.,4.5));
#24733=CARTESIAN_POINT('Origin',(-0.5,62.,0.));
#24734=CARTESIAN_POINT('',(-0.5,31.,58.1935750346352));
#24735=CARTESIAN_POINT('Origin',(-0.5,31.,53.6935750346352));
#24736=CARTESIAN_POINT('',(-0.5,-31.,58.1935750346352));
#24737=CARTESIAN_POINT('Origin',(-0.5,-31.,53.6935750346352));
#24738=CARTESIAN_POINT('',(-0.5,-62.,4.50000000000001));
#24739=CARTESIAN_POINT('Origin',(-0.5,-62.,7.59281015471359E-15));
#24740=CARTESIAN_POINT('',(-0.5,31.,-49.1935750346352));
#24741=CARTESIAN_POINT('Origin',(-0.5,31.,-53.6935750346352));
#24742=CARTESIAN_POINT('',(-0.5,-8.05,-9.85840673313619E-16));
#24743=CARTESIAN_POINT('Origin',(-0.5,0.,0.));
#24744=CARTESIAN_POINT('Origin',(-14.,-72.,30.));
#24745=CARTESIAN_POINT('',(-20.9,-60.,30.));
#24746=CARTESIAN_POINT('',(-20.9,-72.,30.));
#24747=CARTESIAN_POINT('Origin',(-14.,-60.,30.));
#24748=CARTESIAN_POINT('Origin',(-14.,-60.,30.));
#24749=CARTESIAN_POINT('Origin',(-0.4,-31.,-53.6935750346352));
#24750=CARTESIAN_POINT('',(-35.5,-31.,-49.1935750346352));
#24751=CARTESIAN_POINT('',(-0.4,-31.,-49.1935750346352));
#24752=CARTESIAN_POINT('Origin',(-35.5,-31.,-53.6935750346352));
#24753=CARTESIAN_POINT('Origin',(-0.4,62.,0.));
#24754=CARTESIAN_POINT('',(-35.5,62.,4.5));
#24755=CARTESIAN_POINT('',(-0.4,62.,4.5));
#24756=CARTESIAN_POINT('Origin',(-35.5,62.,0.));
#24757=CARTESIAN_POINT('Origin',(-0.4,31.,53.6935750346352));
#24758=CARTESIAN_POINT('',(-35.5,31.,58.1935750346352));
#24759=CARTESIAN_POINT('',(-0.4,31.,58.1935750346352));
#24760=CARTESIAN_POINT('Origin',(-35.5,31.,53.6935750346352));
#24761=CARTESIAN_POINT('Origin',(-0.4,-31.,53.6935750346352));
#24762=CARTESIAN_POINT('',(-35.5,-31.,58.1935750346352));
#24763=CARTESIAN_POINT('',(-0.4,-31.,58.1935750346352));
#24764=CARTESIAN_POINT('Origin',(-35.5,-31.,53.6935750346352));
#24765=CARTESIAN_POINT('Origin',(-0.4,-62.,7.59281015471359E-15));
#24766=CARTESIAN_POINT('',(-35.5,-62.,4.50000000000001));
#24767=CARTESIAN_POINT('',(-0.4,-62.,4.50000000000001));
#24768=CARTESIAN_POINT('Origin',(-35.5,-62.,7.59281015471359E-15));
#24769=CARTESIAN_POINT('Origin',(-0.4,31.,-53.6935750346352));
#24770=CARTESIAN_POINT('',(-35.5,31.,-49.1935750346352));
#24771=CARTESIAN_POINT('',(-0.4,31.,-49.1935750346352));
#24772=CARTESIAN_POINT('Origin',(-35.5,31.,-53.6935750346352));
#24773=CARTESIAN_POINT('Origin',(-20.,35.,0.));
#24774=CARTESIAN_POINT('',(-20.,-35.,-4.28626379701574E-15));
#24775=CARTESIAN_POINT('Origin',(-20.,0.,0.));
#24776=CARTESIAN_POINT('',(-20.,-8.05,-9.85840673313619E-16));
#24777=CARTESIAN_POINT('Origin',(-20.,0.,0.));
#24778=CARTESIAN_POINT('Origin',(-23.,0.,0.));
#24779=CARTESIAN_POINT('',(-26.,-45.,-5.51091059616309E-15));
#24780=CARTESIAN_POINT('',(-23.,-40.,-4.89858719658941E-15));
#24781=CARTESIAN_POINT('Origin',(-26.,0.,0.));
#24782=CARTESIAN_POINT('Origin',(-30.75,0.,0.));
#24783=CARTESIAN_POINT('',(-35.5,-50.,-6.12323399573677E-15));
#24784=CARTESIAN_POINT('',(-30.75,-47.5,-5.81707229594993E-15));
#24785=CARTESIAN_POINT('Origin',(-35.5,0.,0.));
#24786=CARTESIAN_POINT('Origin',(-35.5,69.,0.));
#24787=CARTESIAN_POINT('',(-35.5,-69.,-8.45006291411674E-15));
#24788=CARTESIAN_POINT('Origin',(-35.5,0.,0.));
#24789=CARTESIAN_POINT('Origin',(-35.,0.,0.));
#24790=CARTESIAN_POINT('',(-35.,-69.5,-8.51129525407411E-15));
#24791=CARTESIAN_POINT('Origin',(-10.25,0.,0.));
#24792=CARTESIAN_POINT('',(-10.25,-8.05,-9.85840673313619E-16));
#56598=UNCERTAINTY_MEASURE_WITH_UNIT(LENGTH_MEASURE(0.01),#56640,
'DISTANCE_ACCURACY_VALUE',
'Maximum model space distance between geometric entities at asserted c
onnectivities');
#56617=UNCERTAINTY_MEASURE_WITH_UNIT(LENGTH_MEASURE(0.01),#56640,
'DISTANCE_ACCURACY_VALUE',
'Maximum model space distance between geometric entities at asserted c
onnectivities');
#56620=(
GEOMETRIC_REPRESENTATION_CONTEXT(3)
GLOBAL_UNCERTAINTY_ASSIGNED_CONTEXT((#56598))
GLOBAL_UNIT_ASSIGNED_CONTEXT((#56640,#56642,#56643))
REPRESENTATION_CONTEXT('','3D')
);
#56639=(
GEOMETRIC_REPRESENTATION_CONTEXT(3)
GLOBAL_UNCERTAINTY_ASSIGNED_CONTEXT((#56617))
GLOBAL_UNIT_ASSIGNED_CONTEXT((#56640,#56642,#56643))
REPRESENTATION_CONTEXT('','3D')
);
#56640=(
LENGTH_UNIT()
NAMED_UNIT(*)
SI_UNIT(.MILLI.,.METRE.)
);
#56642=(
NAMED_UNIT(*)
PLANE_ANGLE_UNIT()
SI_UNIT($,.RADIAN.)
);
#56643=(
NAMED_UNIT(*)
SI_UNIT($,.STERADIAN.)
SOLID_ANGLE_UNIT()
);
#56646=SHAPE_DEFINITION_REPRESENTATION(#56667,#56746);
#56667=PRODUCT_DEFINITION_SHAPE('',$,#56768);
#56746=SHAPE_REPRESENTATION('',(#17485),#56620);
#56765=PRODUCT_DEFINITION_CONTEXT('part definition',#56830,'design');
#56768=PRODUCT_DEFINITION('2026-10-26-00-02-39-148',
'02_Center_Body_A_Air_Inlet',#56789,#56765);
#56789=PRODUCT_DEFINITION_FORMATION('',$,#56834);
#56830=APPLICATION_CONTEXT(
'Core Data for Automotive Mechanical Design Process');
#56831=PRODUCT_CONTEXT('part definition',#56830,'mechanical');
#56834=PRODUCT('2026-10-26-00-02-39-148','02_Center_Body_A_Air_Inlet',$,
(#56831));
#56888=COLOUR_RGB('Dark Blue',0.08,0.2,0.34);
#56889=FILL_AREA_STYLE_COLOUR('',#56888);
#56890=FILL_AREA_STYLE('',(#56889));
#56891=SURFACE_STYLE_FILL_AREA(#56890);
#56892=SURFACE_SIDE_STYLE('',(#56891));
#56893=SURFACE_STYLE_USAGE(.BOTH.,#56892);
#56894=PRESENTATION_STYLE_ASSIGNMENT((#56893));
ENDSEC;
END-ISO-10303-21;
